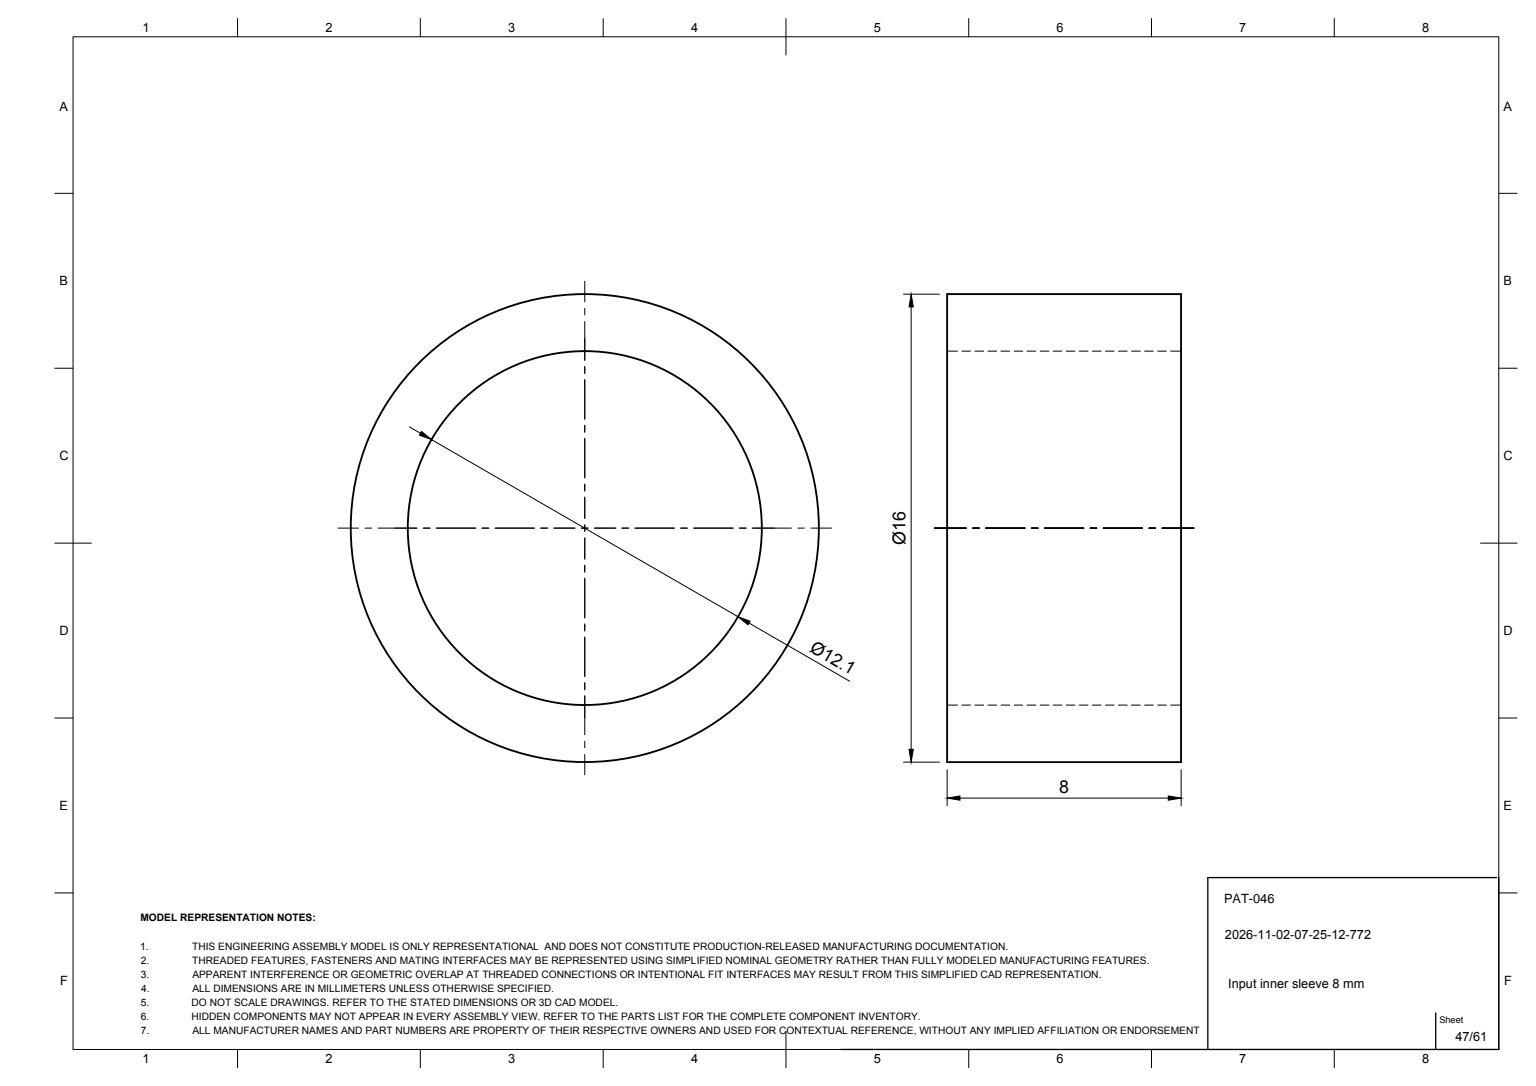
ISO-10303-21;
HEADER;
/* Generated by software containing ST-Developer
 * from STEP Tools, Inc. (www.steptools.com) 
 */

FILE_DESCRIPTION(
/* description */ ('Gear mesh backlash fixture'),
/* implementation_level */ '2;1');

FILE_NAME(
/* name */ 'Input inner sleeve 8 mm.step',
/* time_stamp */ '2026-10-28T03:26:00-07:00',
/* author */ (''),
/* organization */ (''),
/* preprocessor_version */ 'ST-DEVELOPER v20.2',
/* originating_system */ 'Autodesk Translation Framework v15.17.0.0',
/* authorisation */ '');

FILE_SCHEMA (('AUTOMOTIVE_DESIGN { 1 0 10303 214 3 1 1 }'));
ENDSEC;

DATA;
#10=MECHANICAL_DESIGN_GEOMETRIC_PRESENTATION_REPRESENTATION('',(#1066),#57900);
#951=SHAPE_REPRESENTATION_RELATIONSHIP('SRR','None',#58151,#1001);
#1001=ADVANCED_BREP_SHAPE_REPRESENTATION('',(#1129),#57884);
#1066=STYLED_ITEM('',(#58458),#1129);
#1129=MANIFOLD_SOLID_BREP('Body1',#13628);
#1297=FACE_BOUND('',#3035,.T.);
#1298=FACE_BOUND('',#3037,.T.);
#1561=PLANE('',#15083);
#1562=PLANE('',#15084);
#2113=FACE_OUTER_BOUND('',#3032,.T.);
#2114=FACE_OUTER_BOUND('',#3033,.T.);
#2115=FACE_OUTER_BOUND('',#3034,.T.);
#2116=FACE_OUTER_BOUND('',#3036,.T.);
#3032=EDGE_LOOP('',(#10747,#10748,#10749,#10750));
#3033=EDGE_LOOP('',(#10751,#10752,#10753,#10754));
#3034=EDGE_LOOP('',(#10755));
#3035=EDGE_LOOP('',(#10756));
#3036=EDGE_LOOP('',(#10757));
#3037=EDGE_LOOP('',(#10758));
#3895=LINE('',#22074,#4784);
#3896=LINE('',#22080,#4785);
#4784=VECTOR('',#17830,0.605);
#4785=VECTOR('',#17837,0.8);
#5596=CIRCLE('',#15078,0.605);
#5597=CIRCLE('',#15079,0.605);
#5598=CIRCLE('',#15081,0.8);
#5599=CIRCLE('',#15082,0.8);
#6414=VERTEX_POINT('',#22071);
#6415=VERTEX_POINT('',#22073);
#6416=VERTEX_POINT('',#22077);
#6417=VERTEX_POINT('',#22079);
#7960=EDGE_CURVE('',#6414,#6414,#5596,.T.);
#7961=EDGE_CURVE('',#6414,#6415,#3895,.T.);
#7962=EDGE_CURVE('',#6415,#6415,#5597,.T.);
#7963=EDGE_CURVE('',#6416,#6416,#5598,.T.);
#7964=EDGE_CURVE('',#6416,#6417,#3896,.T.);
#7965=EDGE_CURVE('',#6417,#6417,#5599,.T.);
#10747=ORIENTED_EDGE('',*,*,#7960,.F.);
#10748=ORIENTED_EDGE('',*,*,#7961,.T.);
#10749=ORIENTED_EDGE('',*,*,#7962,.T.);
#10750=ORIENTED_EDGE('',*,*,#7961,.F.);
#10751=ORIENTED_EDGE('',*,*,#7963,.F.);
#10752=ORIENTED_EDGE('',*,*,#7964,.T.);
#10753=ORIENTED_EDGE('',*,*,#7965,.T.);
#10754=ORIENTED_EDGE('',*,*,#7964,.F.);
#10755=ORIENTED_EDGE('',*,*,#7963,.T.);
#10756=ORIENTED_EDGE('',*,*,#7960,.T.);
#10757=ORIENTED_EDGE('',*,*,#7965,.F.);
#10758=ORIENTED_EDGE('',*,*,#7962,.F.);
#12722=CYLINDRICAL_SURFACE('',#15077,0.605);
#12723=CYLINDRICAL_SURFACE('',#15080,0.8);
#13230=ADVANCED_FACE('',(#2113),#12722,.F.);
#13231=ADVANCED_FACE('',(#2114),#12723,.T.);
#13232=ADVANCED_FACE('',(#2115,#1297),#1561,.T.);
#13233=ADVANCED_FACE('',(#2116,#1298),#1562,.F.);
#13628=CLOSED_SHELL('',(#13230,#13231,#13232,#13233));
#15076=AXIS2_PLACEMENT_3D('',#22069,#17824,#17825);
#15077=AXIS2_PLACEMENT_3D('',#22070,#17826,#17827);
#15078=AXIS2_PLACEMENT_3D('',#22072,#17828,#17829);
#15079=AXIS2_PLACEMENT_3D('',#22075,#17831,#17832);
#15080=AXIS2_PLACEMENT_3D('',#22076,#17833,#17834);
#15081=AXIS2_PLACEMENT_3D('',#22078,#17835,#17836);
#15082=AXIS2_PLACEMENT_3D('',#22081,#17838,#17839);
#15083=AXIS2_PLACEMENT_3D('',#22082,#17840,#17841);
#15084=AXIS2_PLACEMENT_3D('',#22083,#17842,#17843);
#17824=DIRECTION('axis',(0.,0.,1.));
#17825=DIRECTION('refdir',(1.,0.,0.));
#17826=DIRECTION('center_axis',(0.,0.,1.));
#17827=DIRECTION('ref_axis',(1.,0.,0.));
#17828=DIRECTION('center_axis',(0.,0.,-1.));
#17829=DIRECTION('ref_axis',(1.,0.,0.));
#17830=DIRECTION('',(0.,0.,-1.));
#17831=DIRECTION('center_axis',(0.,0.,-1.));
#17832=DIRECTION('ref_axis',(1.,0.,0.));
#17833=DIRECTION('center_axis',(0.,0.,1.));
#17834=DIRECTION('ref_axis',(1.,0.,0.));
#17835=DIRECTION('center_axis',(0.,0.,1.));
#17836=DIRECTION('ref_axis',(1.,0.,0.));
#17837=DIRECTION('',(0.,0.,-1.));
#17838=DIRECTION('center_axis',(0.,0.,1.));
#17839=DIRECTION('ref_axis',(1.,0.,0.));
#17840=DIRECTION('center_axis',(0.,0.,1.));
#17841=DIRECTION('ref_axis',(1.,0.,0.));
#17842=DIRECTION('center_axis',(0.,0.,1.));
#17843=DIRECTION('ref_axis',(1.,0.,0.));
#22069=CARTESIAN_POINT('',(0.,0.,0.));
#22070=CARTESIAN_POINT('Origin',(0.,0.,14.2));
#22071=CARTESIAN_POINT('',(-0.605,-7.40911313484149E-17,15.));
#22072=CARTESIAN_POINT('Origin',(0.,0.,15.));
#22073=CARTESIAN_POINT('',(-0.605,-7.40911313484149E-17,14.2));
#22074=CARTESIAN_POINT('',(-0.605,-7.40911313484149E-17,14.2));
#22075=CARTESIAN_POINT('Origin',(0.,0.,14.2));
#22076=CARTESIAN_POINT('Origin',(0.,0.,14.2));
#22077=CARTESIAN_POINT('',(-0.8,-9.79717439317883E-17,15.));
#22078=CARTESIAN_POINT('Origin',(0.,0.,15.));
#22079=CARTESIAN_POINT('',(-0.8,-9.79717439317883E-17,14.2));
#22080=CARTESIAN_POINT('',(-0.8,-9.79717439317883E-17,14.2));
#22081=CARTESIAN_POINT('Origin',(0.,0.,14.2));
#22082=CARTESIAN_POINT('Origin',(0.,0.,15.));
#22083=CARTESIAN_POINT('Origin',(0.,0.,14.2));
#57825=UNCERTAINTY_MEASURE_WITH_UNIT(LENGTH_MEASURE(0.001),#57901,
'DISTANCE_ACCURACY_VALUE',
'Maximum model space distance between geometric entities at asserted c
onnectivities');
#57841=UNCERTAINTY_MEASURE_WITH_UNIT(LENGTH_MEASURE(0.001),#57901,
'DISTANCE_ACCURACY_VALUE',
'Maximum model space distance between geometric entities at asserted c
onnectivities');
#57884=(
GEOMETRIC_REPRESENTATION_CONTEXT(3)
GLOBAL_UNCERTAINTY_ASSIGNED_CONTEXT((#57825))
GLOBAL_UNIT_ASSIGNED_CONTEXT((#57901,#57903,#57904))
REPRESENTATION_CONTEXT('','3D')
);
#57900=(
GEOMETRIC_REPRESENTATION_CONTEXT(3)
GLOBAL_UNCERTAINTY_ASSIGNED_CONTEXT((#57841))
GLOBAL_UNIT_ASSIGNED_CONTEXT((#57901,#57903,#57904))
REPRESENTATION_CONTEXT('','3D')
);
#57901=(
LENGTH_UNIT()
NAMED_UNIT(*)
SI_UNIT(.CENTI.,.METRE.)
);
#57903=(
NAMED_UNIT(*)
PLANE_ANGLE_UNIT()
SI_UNIT($,.RADIAN.)
);
#57904=(
NAMED_UNIT(*)
SI_UNIT($,.STERADIAN.)
SOLID_ANGLE_UNIT()
);
#57947=SHAPE_DEFINITION_REPRESENTATION(#58018,#58151);
#58018=PRODUCT_DEFINITION_SHAPE('',$,#58210);
#58151=SHAPE_REPRESENTATION('',(#15076),#57884);
#58167=PRODUCT_DEFINITION_CONTEXT('part definition',#58343,'design');
#58210=PRODUCT_DEFINITION('Input inner sleeve 8 mm',
'Input inner sleeve 8 mm',#58268,#58167);
#58268=PRODUCT_DEFINITION_FORMATION('',$,#58387);
#58343=APPLICATION_CONTEXT(
'Core Data for Automotive Mechanical Design Process');
#58344=PRODUCT_CONTEXT('part definition',#58343,'mechanical');
#58387=PRODUCT('Input inner sleeve 8 mm','Input inner sleeve 8 mm',
'Input inner sleeve 8 mm',(#58344));
#58452=COLOUR_RGB('Sky Blue',0.24,0.69,0.87);
#58453=FILL_AREA_STYLE_COLOUR('',#58452);
#58454=FILL_AREA_STYLE('',(#58453));
#58455=SURFACE_STYLE_FILL_AREA(#58454);
#58456=SURFACE_SIDE_STYLE('',(#58455));
#58457=SURFACE_STYLE_USAGE(.BOTH.,#58456);
#58458=PRESENTATION_STYLE_ASSIGNMENT((#58457));
ENDSEC;
END-ISO-10303-21;
